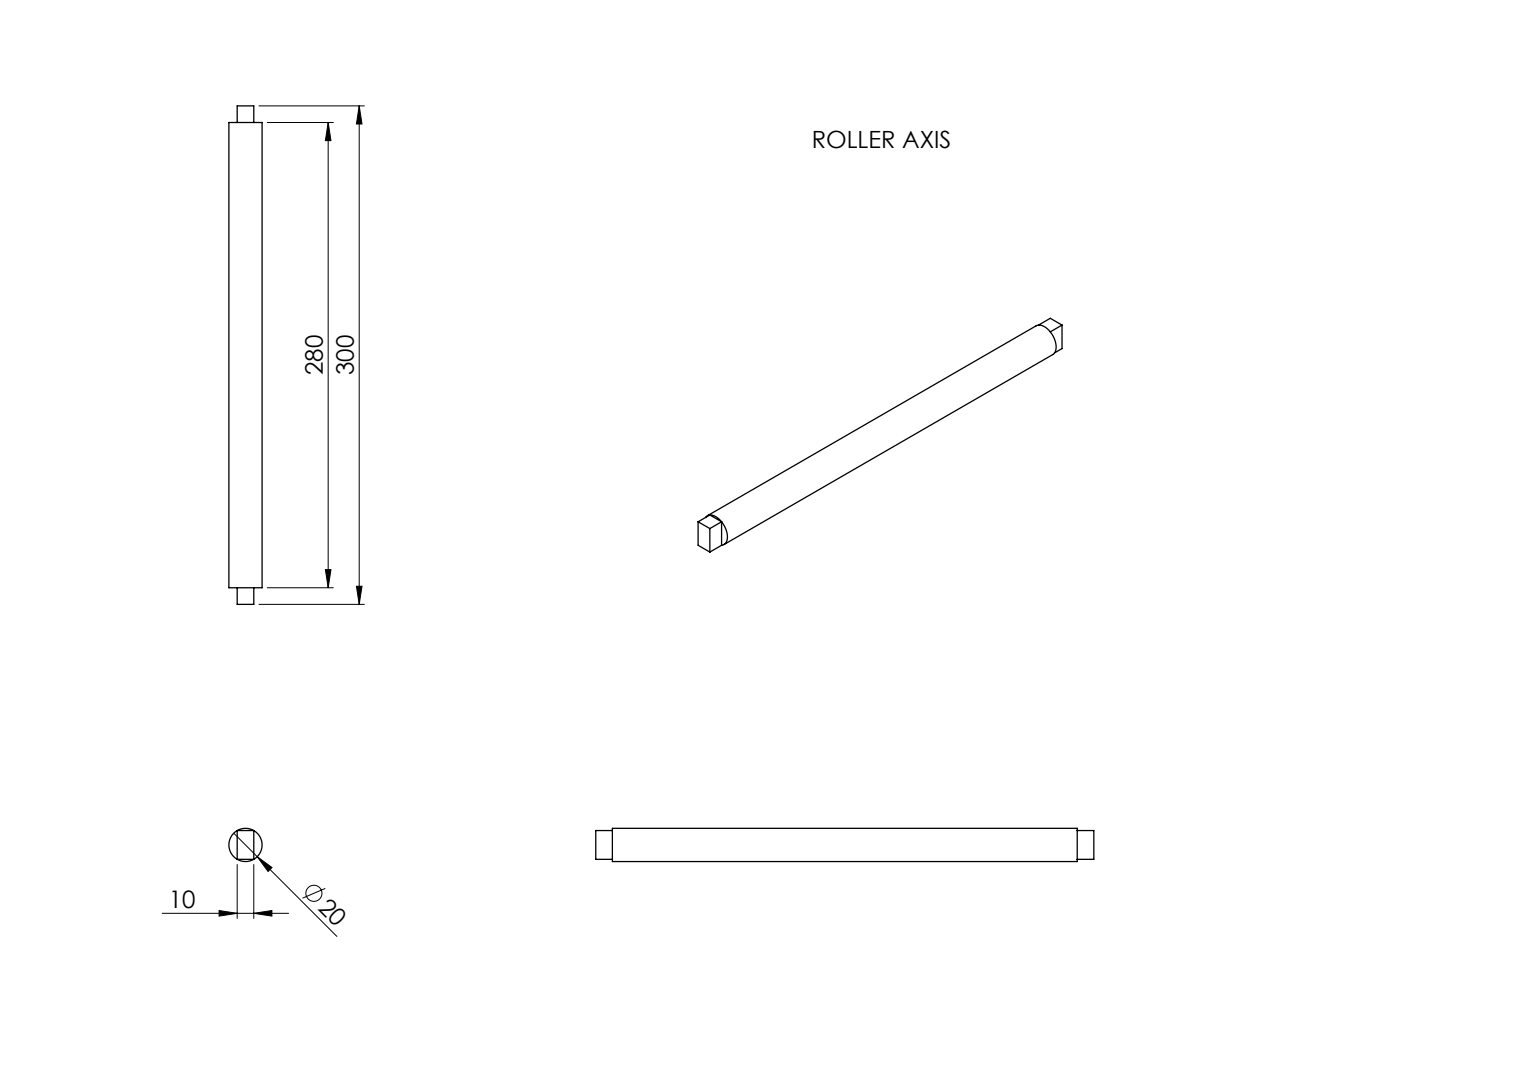
ISO-10303-21;
HEADER;
FILE_DESCRIPTION (('STEP AP214'),
    '1' );
FILE_NAME ('roller axis.step',
    '2026-10-24T14:05:44',
    ( '' ),
    ( '' ),
    'SwSTEP 2.0',
    'SolidWorks 2026',
    '' );
FILE_SCHEMA (( 'AUTOMOTIVE_DESIGN' ));
ENDSEC;

DATA;
#12=PLANE ( 'NONE',  #5087 ) ;
#25=ORIENTED_EDGE ( 'NONE', *, *, #1141, .F. ) ;
#27=CARTESIAN_POINT ( 'NONE',  ( 0.000000000000000000, 0.000000000000000000, 140.0000000000000000 ) ) ;
#37=FILL_AREA_STYLE_COLOUR ( '', #3895 ) ;
#41=AXIS2_PLACEMENT_3D ( 'NONE', #7313, #7278, #7239 ) ;
#47=FACE_OUTER_BOUND ( 'NONE', #4847, .T. ) ;
#52=DIRECTION ( 'NONE',  ( 0.000000000000000000, -0.000000000000000000, 1.000000000000000000 ) ) ;
#53=CARTESIAN_POINT ( 'NONE',  ( 4.999999999999997335, -8.660254037844389075, -140.0000000000000000 ) ) ;
#72=ORIENTED_EDGE ( 'NONE', *, *, #5764, .T. ) ;
#80=CARTESIAN_POINT ( 'NONE',  ( -5.000000000000000888, 8.660254037844390851, 150.0000000000000000 ) ) ;
#83=DIRECTION ( 'NONE',  ( 1.000000000000000000, 0.000000000000000000, -0.000000000000000000 ) ) ;
#94=ADVANCED_FACE ( 'NONE', ( #3566 ), #5869, .F. ) ;
#97=DIRECTION ( 'NONE',  ( 1.000000000000000000, 0.000000000000000000, -0.000000000000000000 ) ) ;
#100=LINE ( 'NONE', #5559, #7316 ) ;
#117=PLANE ( 'NONE',  #3650 ) ;
#124=ORIENTED_EDGE ( 'NONE', *, *, #2636, .T. ) ;
#128=PLANE ( 'NONE',  #3351 ) ;
#140=EDGE_LOOP ( 'NONE', ( #451, #3034, #5054, #639, #3841, #3880, #6414, #6214 ) ) ;
#149=CARTESIAN_POINT ( 'NONE',  ( -5.000000000000000888, -8.660254037844389075, -150.0000000000000000 ) ) ;
#172=DIRECTION ( 'NONE',  ( -1.000000000000000000, 0.000000000000000000, 0.000000000000000000 ) ) ;
#174=ORIENTED_EDGE ( 'NONE', *, *, #1060, .T. ) ;
#181=CIRCLE ( 'NONE', #4359, 10.00000000000000000 ) ;
#189=CARTESIAN_POINT ( 'NONE',  ( 4.999999999999999112, 8.660254037844390851, 150.0000000000000000 ) ) ;
#191=FACE_OUTER_BOUND ( 'NONE', #1286, .T. ) ;
#199=ORIENTED_EDGE ( 'NONE', *, *, #1070, .F. ) ;
#205=ADVANCED_FACE ( 'NONE', ( #4414 ), #1489, .F. ) ;
#217=ORIENTED_EDGE ( 'NONE', *, *, #4171, .T. ) ;
#221=DIRECTION ( 'NONE',  ( 0.000000000000000000, -1.000000000000000000, 0.000000000000000000 ) ) ;
#252=ORIENTED_EDGE ( 'NONE', *, *, #6107, .T. ) ;
#256=AXIS2_PLACEMENT_3D ( 'NONE', #4917, #1432, #2617 ) ;
#292=ORIENTED_EDGE ( 'NONE', *, *, #3168, .F. ) ;
#300=ORIENTED_EDGE ( 'NONE', *, *, #2593, .F. ) ;
#328=DIRECTION ( 'NONE',  ( 1.000000000000000000, 0.000000000000000000, 0.000000000000000000 ) ) ;
#331=ADVANCED_FACE ( 'NONE', ( #6163 ), #6723, .T. ) ;
#352=CYLINDRICAL_SURFACE ( 'NONE', #41, 10.00000000000000000 ) ;
#359=DIRECTION ( 'NONE',  ( -0.000000000000000000, -0.000000000000000000, -1.000000000000000000 ) ) ;
#360=ORIENTED_EDGE ( 'NONE', *, *, #1641, .T. ) ;
#363=FACE_OUTER_BOUND ( 'NONE', #5495, .T. ) ;
#384=ORIENTED_EDGE ( 'NONE', *, *, #3152, .F. ) ;
#392=FACE_OUTER_BOUND ( 'NONE', #2164, .T. ) ;
#397=FACE_OUTER_BOUND ( 'NONE', #140, .T. ) ;
#422=CARTESIAN_POINT ( 'NONE',  ( -5.000000000000000888, -8.660254037844389075, -140.0000000000000284 ) ) ;
#424=CARTESIAN_POINT ( 'NONE',  ( -10.00000000000000000, 0.000000000000000000, -140.0000000000000000 ) ) ;
#426=ORIENTED_EDGE ( 'NONE', *, *, #4897, .F. ) ;
#451=ORIENTED_EDGE ( 'NONE', *, *, #5219, .F. ) ;
#454=EDGE_LOOP ( 'NONE', ( #6459, #72, #5565, #1387 ) ) ;
#456=DIRECTION ( 'NONE',  ( 1.000000000000000000, 0.000000000000000000, -0.000000000000000000 ) ) ;
#457=CARTESIAN_POINT ( 'NONE',  ( -5.000000000000000888, 8.660254037844390851, -150.0000000000000000 ) ) ;
#476=ORIENTED_EDGE ( 'NONE', *, *, #4916, .F. ) ;
#477=LINE ( 'NONE', #3366, #540 ) ;
#537=AXIS2_PLACEMENT_3D ( 'NONE', #2124, #3352, #7303 ) ;
#540=VECTOR ( 'NONE', #6836, 1000.000000000000000 ) ;
#568=DIRECTION ( 'NONE',  ( 1.000000000000000000, 0.000000000000000000, 0.000000000000000000 ) ) ;
#569=AXIS2_PLACEMENT_3D ( 'NONE', #2262, #6216, #568 ) ;
#572=CARTESIAN_POINT ( 'NONE',  ( -5.000000000000000888, 8.660254037844390851, 150.0000000000000000 ) ) ;
#590=CARTESIAN_POINT ( 'NONE',  ( 4.999999999999999112, 8.660254037844390851, -150.0000000000000000 ) ) ;
#597=CARTESIAN_POINT ( 'NONE',  ( -5.000000000000000888, 0.000000000000000000, 140.0000000000000000 ) ) ;
#609=LINE ( 'NONE', #1723, #1679 ) ;
#611=CARTESIAN_POINT ( 'NONE',  ( -5.000000000000000888, -8.660254037844389075, 150.0000000000000000 ) ) ;
#613=ADVANCED_FACE ( 'NONE', ( #47 ), #1091, .F. ) ;
#627=ADVANCED_FACE ( 'NONE', ( #4608 ), #12, .F. ) ;
#628=DIRECTION ( 'NONE',  ( 0.000000000000000000, 0.000000000000000000, 1.000000000000000000 ) ) ;
#630=VERTEX_POINT ( 'NONE', #2832 ) ;
#633=CARTESIAN_POINT ( 'NONE',  ( 0.000000000000000000, 0.000000000000000000, 140.0000000000000000 ) ) ;
#634=LINE ( 'NONE', #149, #4836 ) ;
#639=ORIENTED_EDGE ( 'NONE', *, *, #6547, .F. ) ;
#640=AXIS2_PLACEMENT_3D ( 'NONE', #2848, #6942, #1184 ) ;
#650=AXIS2_PLACEMENT_3D ( 'NONE', #2212, #6051, #988 ) ;
#660=EDGE_CURVE ( 'NONE', #6352, #1004, #181, .T. ) ;
#667=EDGE_LOOP ( 'NONE', ( #840, #4739, #1362, #2962 ) ) ;
#670=STYLED_ITEM ( 'NONE', ( #5899 ), #1370 ) ;
#671=ORIENTED_EDGE ( 'NONE', *, *, #5764, .F. ) ;
#689=ORIENTED_EDGE ( 'NONE', *, *, #5366, .F. ) ;
#692=DIRECTION ( 'NONE',  ( 0.000000000000000000, 0.000000000000000000, 1.000000000000000000 ) ) ;
#740=ADVANCED_FACE ( 'NONE', ( #1129 ), #5700, .F. ) ;
#755=AXIS2_PLACEMENT_3D ( 'NONE', #1285, #4088, #6492 ) ;
#783=ORIENTED_EDGE ( 'NONE', *, *, #4897, .T. ) ;
#794=MANIFOLD_SOLID_BREP ( 'Boss-Extrude2', #5074 ) ;
#820=LINE ( 'NONE', #2560, #5650 ) ;
#832=ADVANCED_FACE ( 'NONE', ( #191 ), #117, .T. ) ;
#840=ORIENTED_EDGE ( 'NONE', *, *, #4441, .F. ) ;
#862=CARTESIAN_POINT ( 'NONE',  ( 0.000000000000000000, 0.000000000000000000, 150.0000000000000000 ) ) ;
#876=CARTESIAN_POINT ( 'NONE',  ( 0.000000000000000000, 8.660254037844390851, -140.0000000000000000 ) ) ;
#901=CARTESIAN_POINT ( 'NONE',  ( 10.00000000000000000, 1.224646799147353256E-15, 140.0000000000000000 ) ) ;
#907=PLANE ( 'NONE',  #5104 ) ;
#919=DIRECTION ( 'NONE',  ( 1.000000000000000000, 0.000000000000000000, -0.000000000000000000 ) ) ;
#942=ORIENTED_EDGE ( 'NONE', *, *, #5085, .T. ) ;
#944=CARTESIAN_POINT ( 'NONE',  ( 4.999999999999999112, 8.660254037844390851, 150.0000000000000000 ) ) ;
#981=ORIENTED_EDGE ( 'NONE', *, *, #1995, .F. ) ;
#988=DIRECTION ( 'NONE',  ( 1.000000000000000000, 0.000000000000000000, -0.000000000000000000 ) ) ;
#1004=VERTEX_POINT ( 'NONE', #5611 ) ;
#1008=AXIS2_PLACEMENT_3D ( 'NONE', #4801, #1517, #3094 ) ;
#1051=CARTESIAN_POINT ( 'NONE',  ( 4.999999999999999112, 8.660254037844390851, -150.0000000000000000 ) ) ;
#1060=EDGE_CURVE ( 'NONE', #6894, #5855, #4448, .T. ) ;
#1070=EDGE_CURVE ( 'NONE', #6814, #1780, #4561, .T. ) ;
#1073=EDGE_CURVE ( 'NONE', #7081, #5227, #4988, .T. ) ;
#1083=CARTESIAN_POINT ( 'NONE',  ( 4.999999999999999112, 0.000000000000000000, 140.0000000000000000 ) ) ;
#1091=PLANE ( 'NONE',  #6280 ) ;
#1094=EDGE_CURVE ( 'NONE', #6847, #3802, #5018, .T. ) ;
#1098=DIRECTION ( 'NONE',  ( 1.000000000000000000, 0.000000000000000000, -0.000000000000000000 ) ) ;
#1112=VECTOR ( 'NONE', #5415, 1000.000000000000000 ) ;
#1129=FACE_OUTER_BOUND ( 'NONE', #1317, .T. ) ;
#1132=ORIENTED_EDGE ( 'NONE', *, *, #7005, .F. ) ;
#1141=EDGE_CURVE ( 'NONE', #4157, #630, #4032, .T. ) ;
#1178=CARTESIAN_POINT ( 'NONE',  ( -5.000000000000000888, 8.660254037844390851, 150.0000000000000000 ) ) ;
#1184=DIRECTION ( 'NONE',  ( 1.000000000000000000, 0.000000000000000000, 0.000000000000000000 ) ) ;
#1189=EDGE_CURVE ( 'NONE', #2308, #3238, #6358, .T. ) ;
#1193=SHAPE_REPRESENTATION ( 'roller axis', ( #1963 ), #5205 ) ;
#1199=DIRECTION ( 'NONE',  ( 0.000000000000000000, -1.000000000000000000, 0.000000000000000000 ) ) ;
#1204=FACE_OUTER_BOUND ( 'NONE', #2091, .T. ) ;
#1208=LINE ( 'NONE', #1178, #5962 ) ;
#1219=ORIENTED_EDGE ( 'NONE', *, *, #1141, .T. ) ;
#1228=DIRECTION ( 'NONE',  ( 0.000000000000000000, -0.000000000000000000, 1.000000000000000000 ) ) ;
#1249=LINE ( 'NONE', #6980, #6621 ) ;
#1285=CARTESIAN_POINT ( 'NONE',  ( 0.000000000000000000, 0.000000000000000000, -140.0000000000000000 ) ) ;
#1286=EDGE_LOOP ( 'NONE', ( #2523, #5606 ) ) ;
#1294=CARTESIAN_POINT ( 'NONE',  ( -5.000000000000000888, -8.660254037844389075, 150.0000000000000000 ) ) ;
#1299=DIRECTION ( 'NONE',  ( 0.000000000000000000, 1.000000000000000000, 0.000000000000000000 ) ) ;
#1317=EDGE_LOOP ( 'NONE', ( #6784, #6485, #783, #2163 ) ) ;
#1327=ORIENTED_EDGE ( 'NONE', *, *, #2416, .F. ) ;
#1329=AXIS2_PLACEMENT_3D ( 'NONE', #611, #5171, #52 ) ;
#1342=PRODUCT_DEFINITION_SHAPE ( 'NONE', 'NONE',  #6666 ) ;
#1352=ADVANCED_FACE ( 'NONE', ( #363 ), #4845, .F. ) ;
#1362=ORIENTED_EDGE ( 'NONE', *, *, #6828, .F. ) ;
#1364=EDGE_CURVE ( 'NONE', #2884, #6814, #4018, .T. ) ;
#1370=ADVANCED_BREP_SHAPE_REPRESENTATION ( '', ( #794, #1963 ), #5205 ) ;
#1376=( NAMED_UNIT ( * ) SI_UNIT ( $, .STERADIAN. ) SOLID_ANGLE_UNIT ( ) );
#1385=VECTOR ( 'NONE', #6183, 1000.000000000000000 ) ;
#1387=ORIENTED_EDGE ( 'NONE', *, *, #4449, .T. ) ;
#1432=DIRECTION ( 'NONE',  ( -0.000000000000000000, -0.000000000000000000, -1.000000000000000000 ) ) ;
#1471=CARTESIAN_POINT ( 'NONE',  ( -5.000000000000000888, -8.660254037844389075, 150.0000000000000000 ) ) ;
#1489=PLANE ( 'NONE',  #5904 ) ;
#1517=DIRECTION ( 'NONE',  ( 0.000000000000000000, 0.000000000000000000, 1.000000000000000000 ) ) ;
#1542=CARTESIAN_POINT ( 'NONE',  ( -5.000000000000000888, -8.660254037844389075, 150.0000000000000000 ) ) ;
#1548=CARTESIAN_POINT ( 'NONE',  ( 0.000000000000000000, 0.000000000000000000, -150.0000000000000000 ) ) ;
#1550=VERTEX_POINT ( 'NONE', #3299 ) ;
#1553=DIRECTION ( 'NONE',  ( 0.000000000000000000, -1.000000000000000000, 0.000000000000000000 ) ) ;
#1560=ORIENTED_EDGE ( 'NONE', *, *, #1073, .F. ) ;
#1570=PLANE ( 'NONE',  #537 ) ;
#1641=EDGE_CURVE ( 'NONE', #6814, #630, #6528, .T. ) ;
#1648=ORIENTED_EDGE ( 'NONE', *, *, #3152, .T. ) ;
#1679=VECTOR ( 'NONE', #4012, 1000.000000000000000 ) ;
#1719=CARTESIAN_POINT ( 'NONE',  ( -5.000000000000000888, -8.660254037844389075, 150.0000000000000000 ) ) ;
#1723=CARTESIAN_POINT ( 'NONE',  ( 10.00000000000000000, 1.224646799147353256E-15, 140.0000000000000000 ) ) ;
#1727=VECTOR ( 'NONE', #5465, 1000.000000000000000 ) ;
#1735=DIRECTION ( 'NONE',  ( 0.000000000000000000, 0.000000000000000000, 1.000000000000000000 ) ) ;
#1743=ADVANCED_FACE ( 'NONE', ( #4907 ), #907, .T. ) ;
#1747=( NAMED_UNIT ( * ) SI_UNIT ( $, .STERADIAN. ) SOLID_ANGLE_UNIT ( ) );
#1760=PLANE ( 'NONE',  #4967 ) ;
#1765=DIRECTION ( 'NONE',  ( 1.000000000000000000, 0.000000000000000000, 0.000000000000000000 ) ) ;
#1780=VERTEX_POINT ( 'NONE', #4271 ) ;
#1911=ORIENTED_EDGE ( 'NONE', *, *, #6967, .T. ) ;
#1963=AXIS2_PLACEMENT_3D ( 'NONE', #2294, #628, #5829 ) ;
#1989=DIRECTION ( 'NONE',  ( 1.000000000000000000, 0.000000000000000000, -0.000000000000000000 ) ) ;
#1994=CARTESIAN_POINT ( 'NONE',  ( 4.999999999999999112, -8.660254037844389075, -150.0000000000000000 ) ) ;
#1995=EDGE_CURVE ( 'NONE', #5227, #6735, #2563, .T. ) ;
#2008=ORIENTED_EDGE ( 'NONE', *, *, #5138, .T. ) ;
#2091=EDGE_LOOP ( 'NONE', ( #5202, #2859, #2616, #7285 ) ) ;
#2115=EDGE_LOOP ( 'NONE', ( #6569, #2579, #4972 ) ) ;
#2124=CARTESIAN_POINT ( 'NONE',  ( -5.000000000000000888, 8.660254037844390851, 150.0000000000000000 ) ) ;
#2163=ORIENTED_EDGE ( 'NONE', *, *, #7005, .T. ) ;
#2164=EDGE_LOOP ( 'NONE', ( #671, #1560 ) ) ;
#2206=LINE ( 'NONE', #7310, #2963 ) ;
#2212=CARTESIAN_POINT ( 'NONE',  ( 0.000000000000000000, 0.000000000000000000, 140.0000000000000000 ) ) ;
#2246=DIRECTION ( 'NONE',  ( 0.000000000000000000, 0.000000000000000000, 1.000000000000000000 ) ) ;
#2262=CARTESIAN_POINT ( 'NONE',  ( 0.000000000000000000, 0.000000000000000000, -140.0000000000000000 ) ) ;
#2274=DIRECTION ( 'NONE',  ( 0.000000000000000000, 0.000000000000000000, 1.000000000000000000 ) ) ;
#2277=CARTESIAN_POINT ( 'NONE',  ( 0.000000000000000000, 0.000000000000000000, -140.0000000000000000 ) ) ;
#2282=ORIENTED_EDGE ( 'NONE', *, *, #4441, .T. ) ;
#2289=EDGE_CURVE ( 'NONE', #6735, #5434, #5541, .T. ) ;
#2293=ORIENTED_EDGE ( 'NONE', *, *, #1094, .F. ) ;
#2294=CARTESIAN_POINT ( 'NONE',  ( 0.000000000000000000, 0.000000000000000000, 0.000000000000000000 ) ) ;
#2308=VERTEX_POINT ( 'NONE', #1471 ) ;
#2349=ORIENTED_EDGE ( 'NONE', *, *, #1070, .T. ) ;
#2400=DIRECTION ( 'NONE',  ( 1.000000000000000000, 0.000000000000000000, -0.000000000000000000 ) ) ;
#2416=EDGE_CURVE ( 'NONE', #1550, #6735, #5364, .T. ) ;
#2426=DIRECTION ( 'NONE',  ( 0.000000000000000000, 0.000000000000000000, 1.000000000000000000 ) ) ;
#2469=PRODUCT ( 'roller axis', 'roller axis', '', ( #3485 ) ) ;
#2487=ADVANCED_FACE ( 'NONE', ( #392 ), #6052, .F. ) ;
#2518=EDGE_LOOP ( 'NONE', ( #360, #2282 ) ) ;
#2522=DIRECTION ( 'NONE',  ( 0.000000000000000000, 0.000000000000000000, 1.000000000000000000 ) ) ;
#2523=ORIENTED_EDGE ( 'NONE', *, *, #3458, .T. ) ;
#2541=ADVANCED_FACE ( 'NONE', ( #6567 ), #7199, .F. ) ;
#2560=CARTESIAN_POINT ( 'NONE',  ( 0.000000000000000000, -8.660254037844389075, -140.0000000000000000 ) ) ;
#2563=CIRCLE ( 'NONE', #3526, 10.00000000000000000 ) ;
#2579=ORIENTED_EDGE ( 'NONE', *, *, #6613, .F. ) ;
#2593=EDGE_CURVE ( 'NONE', #2887, #6814, #477, .T. ) ;
#2598=DIRECTION ( 'NONE',  ( -1.000000000000000000, 0.000000000000000000, 0.000000000000000000 ) ) ;
#2601=DIRECTION ( 'NONE',  ( 1.000000000000000000, 0.000000000000000000, 0.000000000000000000 ) ) ;
#2616=ORIENTED_EDGE ( 'NONE', *, *, #1189, .F. ) ;
#2617=DIRECTION ( 'NONE',  ( -1.000000000000000000, 0.000000000000000000, 0.000000000000000000 ) ) ;
#2624=CARTESIAN_POINT ( 'NONE',  ( -5.000000000000000888, 8.660254037844390851, 150.0000000000000000 ) ) ;
#2631=LINE ( 'NONE', #7140, #5691 ) ;
#2636=EDGE_CURVE ( 'NONE', #5227, #6847, #1208, .T. ) ;
#2648=LINE ( 'NONE', #1542, #2756 ) ;
#2686=VECTOR ( 'NONE', #2828, 1000.000000000000000 ) ;
#2693=EDGE_LOOP ( 'NONE', ( #6432, #7023, #1911, #5734 ) ) ;
#2700=DIRECTION ( 'NONE',  ( 1.000000000000000000, 0.000000000000000000, -0.000000000000000000 ) ) ;
#2739=CARTESIAN_POINT ( 'NONE',  ( 0.000000000000000000, 0.000000000000000000, 140.0000000000000000 ) ) ;
#2742=LINE ( 'NONE', #876, #4439 ) ;
#2756=VECTOR ( 'NONE', #4425, 1000.000000000000000 ) ;
#2761=CARTESIAN_POINT ( 'NONE',  ( 0.000000000000000000, 0.000000000000000000, -140.0000000000000000 ) ) ;
#2790=DIRECTION ( 'NONE',  ( 0.000000000000000000, -1.000000000000000000, 0.000000000000000000 ) ) ;
#2828=DIRECTION ( 'NONE',  ( -1.000000000000000000, -0.000000000000000000, -0.000000000000000000 ) ) ;
#2832=CARTESIAN_POINT ( 'NONE',  ( -5.000000000000000888, 8.660254037844390851, 140.0000000000000000 ) ) ;
#2848=CARTESIAN_POINT ( 'NONE',  ( 0.000000000000000000, 0.000000000000000000, 140.0000000000000000 ) ) ;
#2852=DIRECTION ( 'NONE',  ( 0.000000000000000000, -1.000000000000000000, 0.000000000000000000 ) ) ;
#2856=CARTESIAN_POINT ( 'NONE',  ( -5.000000000000000888, 8.660254037844390851, -150.0000000000000000 ) ) ;
#2859=ORIENTED_EDGE ( 'NONE', *, *, #6351, .F. ) ;
#2860=DIRECTION ( 'NONE',  ( -1.000000000000000000, 0.000000000000000000, 0.000000000000000000 ) ) ;
#2863=ORIENTED_EDGE ( 'NONE', *, *, #6967, .F. ) ;
#2865=CARTESIAN_POINT ( 'NONE',  ( -5.000000000000000888, 8.660254037844387298, -140.0000000000000000 ) ) ;
#2884=VERTEX_POINT ( 'NONE', #901 ) ;
#2887=VERTEX_POINT ( 'NONE', #5536 ) ;
#2893=DIRECTION ( 'NONE',  ( 1.000000000000000000, 0.000000000000000000, 0.000000000000000000 ) ) ;
#2897=EDGE_LOOP ( 'NONE', ( #1648, #6143, #1219 ) ) ;
#2906=MECHANICAL_DESIGN_GEOMETRIC_PRESENTATION_REPRESENTATION('',(#670),#4713);
#2962=ORIENTED_EDGE ( 'NONE', *, *, #2593, .T. ) ;
#2963=VECTOR ( 'NONE', #6309, 1000.000000000000000 ) ;
#2979=AXIS2_PLACEMENT_3D ( 'NONE', #2739, #1735, #4517 ) ;
#3034=ORIENTED_EDGE ( 'NONE', *, *, #5138, .F. ) ;
#3037=VECTOR ( 'NONE', #6952, 1000.000000000000000 ) ;
#3094=DIRECTION ( 'NONE',  ( 1.000000000000000000, 0.000000000000000000, 0.000000000000000000 ) ) ;
#3115=ORIENTED_EDGE ( 'NONE', *, *, #1364, .F. ) ;
#3124=VECTOR ( 'NONE', #359, 1000.000000000000000 ) ;
#3150=AXIS2_PLACEMENT_3D ( 'NONE', #2624, #1989, #6063 ) ;
#3152=EDGE_CURVE ( 'NONE', #630, #1550, #5065, .T. ) ;
#3167=CARTESIAN_POINT ( 'NONE',  ( 0.000000000000000000, 0.000000000000000000, -140.0000000000000000 ) ) ;
#3168=EDGE_CURVE ( 'NONE', #3238, #2887, #6917, .T. ) ;
#3188=LINE ( 'NONE', #4294, #1112 ) ;
#3232=EDGE_CURVE ( 'NONE', #5434, #6352, #4697, .T. ) ;
#3238=VERTEX_POINT ( 'NONE', #7022 ) ;
#3273=EDGE_CURVE ( 'NONE', #1780, #4157, #1249, .T. ) ;
#3299=CARTESIAN_POINT ( 'NONE',  ( -10.00000000000000000, 0.000000000000000000, 140.0000000000000000 ) ) ;
#3336=CARTESIAN_POINT ( 'NONE',  ( -4.999999999999997335, -8.660254037844389075, 140.0000000000000000 ) ) ;
#3351=AXIS2_PLACEMENT_3D ( 'NONE', #5322, #97, #3515 ) ;
#3352=DIRECTION ( 'NONE',  ( 0.000000000000000000, -1.000000000000000000, 0.000000000000000000 ) ) ;
#3366=CARTESIAN_POINT ( 'NONE',  ( 4.999999999999999112, 8.660254037844390851, 150.0000000000000000 ) ) ;
#3439=PLANE ( 'NONE',  #1329 ) ;
#3443=DIRECTION ( 'NONE',  ( -0.000000000000000000, -0.000000000000000000, -1.000000000000000000 ) ) ;
#3454=SURFACE_STYLE_FILL_AREA ( #3561 ) ;
#3458=EDGE_CURVE ( 'NONE', #4157, #1780, #7202, .T. ) ;
#3471=PLANE ( 'NONE',  #4280 ) ;
#3485=PRODUCT_CONTEXT ( 'NONE', #3717, 'mechanical' ) ;
#3491=PLANE ( 'NONE',  #6961 ) ;
#3515=DIRECTION ( 'NONE',  ( -0.000000000000000000, 0.000000000000000000, -1.000000000000000000 ) ) ;
#3526=AXIS2_PLACEMENT_3D ( 'NONE', #4013, #5140, #5841 ) ;
#3528=ORIENTED_EDGE ( 'NONE', *, *, #2289, .F. ) ;
#3561=FILL_AREA_STYLE ('',( #37 ) ) ;
#3566=FACE_OUTER_BOUND ( 'NONE', #6734, .T. ) ;
#3567=( NAMED_UNIT ( * ) PLANE_ANGLE_UNIT ( ) SI_UNIT ( $, .RADIAN. ) );
#3649=ADVANCED_FACE ( 'NONE', ( #3700 ), #352, .T. ) ;
#3650=AXIS2_PLACEMENT_3D ( 'NONE', #4177, #6364, #83 ) ;
#3700=FACE_OUTER_BOUND ( 'NONE', #4683, .T. ) ;
#3717=APPLICATION_CONTEXT ( 'automotive_design' ) ;
#3774=VECTOR ( 'NONE', #2852, 1000.000000000000000 ) ;
#3802=VERTEX_POINT ( 'NONE', #4509 ) ;
#3822=CARTESIAN_POINT ( 'NONE',  ( -5.000000000000000888, 0.000000000000000000, -140.0000000000000000 ) ) ;
#3824=DIRECTION ( 'NONE',  ( 1.000000000000000000, 0.000000000000000000, 0.000000000000000000 ) ) ;
#3834=ADVANCED_FACE ( 'NONE', ( #1204 ), #3439, .F. ) ;
#3841=ORIENTED_EDGE ( 'NONE', *, *, #2416, .T. ) ;
#3872=PRODUCT_DEFINITION_FORMATION_WITH_SPECIFIED_SOURCE ( 'ANY', '', #2469, .NOT_KNOWN. ) ;
#3880=ORIENTED_EDGE ( 'NONE', *, *, #2289, .T. ) ;
#3893=CARTESIAN_POINT ( 'NONE',  ( 4.999999999999999112, 8.660254037844390851, 140.0000000000000000 ) ) ;
#3895=COLOUR_RGB ( '',0.8941176470588234615, 0.8941176470588234615, 0.8941176470588234615 ) ;
#3900=ORIENTED_EDGE ( 'NONE', *, *, #1094, .T. ) ;
#3907=FACE_OUTER_BOUND ( 'NONE', #2115, .T. ) ;
#3911=( GEOMETRIC_REPRESENTATION_CONTEXT ( 3 ) GLOBAL_UNCERTAINTY_ASSIGNED_CONTEXT ( ( #4933 ) ) GLOBAL_UNIT_ASSIGNED_CONTEXT ( ( #4749, #3567, #1376 ) ) REPRESENTATION_CONTEXT ( 'NONE', 'WORKASPACE' ) );
#3958=AXIS2_PLACEMENT_3D ( 'NONE', #6227, #2274, #6197 ) ;
#3968=FACE_OUTER_BOUND ( 'NONE', #667, .T. ) ;
#3979=DIRECTION ( 'NONE',  ( -0.000000000000000000, -0.000000000000000000, -1.000000000000000000 ) ) ;
#4008=AXIS2_PLACEMENT_3D ( 'NONE', #6481, #5920, #4077 ) ;
#4012=DIRECTION ( 'NONE',  ( -0.000000000000000000, -0.000000000000000000, -1.000000000000000000 ) ) ;
#4013=CARTESIAN_POINT ( 'NONE',  ( 0.000000000000000000, 0.000000000000000000, -140.0000000000000000 ) ) ;
#4018=CIRCLE ( 'NONE', #5570, 10.00000000000000000 ) ;
#4032=LINE ( 'NONE', #597, #1385 ) ;
#4038=PLANE ( 'NONE',  #2979 ) ;
#4077=DIRECTION ( 'NONE',  ( 1.000000000000000000, 0.000000000000000000, 0.000000000000000000 ) ) ;
#4088=DIRECTION ( 'NONE',  ( 0.000000000000000000, 0.000000000000000000, 1.000000000000000000 ) ) ;
#4110=AXIS2_PLACEMENT_3D ( 'NONE', #1719, #1299, #1228 ) ;
#4138=( LENGTH_UNIT ( ) NAMED_UNIT ( * ) SI_UNIT ( .MILLI., .METRE. ) );
#4157=VERTEX_POINT ( 'NONE', #3336 ) ;
#4171=EDGE_CURVE ( 'NONE', #7081, #6352, #7066, .T. ) ;
#4177=CARTESIAN_POINT ( 'NONE',  ( 0.000000000000000000, 0.000000000000000000, 140.0000000000000000 ) ) ;
#4248=CARTESIAN_POINT ( 'NONE',  ( 0.000000000000000000, 0.000000000000000000, 140.0000000000000000 ) ) ;
#4271=CARTESIAN_POINT ( 'NONE',  ( 4.999999999999999112, -8.660254037844389075, 140.0000000000000000 ) ) ;
#4280=AXIS2_PLACEMENT_3D ( 'NONE', #5771, #2246, #1098 ) ;
#4294=CARTESIAN_POINT ( 'NONE',  ( -5.000000000000000888, -8.660254037844389075, 150.0000000000000000 ) ) ;
#4307=DIRECTION ( 'NONE',  ( 1.000000000000000000, 0.000000000000000000, 0.000000000000000000 ) ) ;
#4315=VECTOR ( 'NONE', #4391, 1000.000000000000000 ) ;
#4331=ORIENTED_EDGE ( 'NONE', *, *, #1364, .T. ) ;
#4344=AXIS2_PLACEMENT_3D ( 'NONE', #189, #4748, #7034 ) ;
#4359=AXIS2_PLACEMENT_3D ( 'NONE', #2761, #6649, #2893 ) ;
#4391=DIRECTION ( 'NONE',  ( -0.000000000000000000, -0.000000000000000000, -1.000000000000000000 ) ) ;
#4398=DIRECTION ( 'NONE',  ( 0.000000000000000000, 0.000000000000000000, 1.000000000000000000 ) ) ;
#4410=ORIENTED_EDGE ( 'NONE', *, *, #5435, .F. ) ;
#4414=FACE_OUTER_BOUND ( 'NONE', #4976, .T. ) ;
#4416=EDGE_LOOP ( 'NONE', ( #2008, #4331, #2349 ) ) ;
#4425=DIRECTION ( 'NONE',  ( -0.000000000000000000, -0.000000000000000000, -1.000000000000000000 ) ) ;
#4433=EDGE_LOOP ( 'NONE', ( #4672, #1132, #2293, #5210 ) ) ;
#4439=VECTOR ( 'NONE', #919, 1000.000000000000000 ) ;
#4440=VECTOR ( 'NONE', #1553, 1000.000000000000000 ) ;
#4441=EDGE_CURVE ( 'NONE', #630, #6814, #6281, .T. ) ;
#4448=LINE ( 'NONE', #1051, #7015 ) ;
#4449=EDGE_CURVE ( 'NONE', #5855, #6847, #100, .T. ) ;
#4475=CARTESIAN_POINT ( 'NONE',  ( 4.999999999999999112, 0.000000000000000000, -140.0000000000000000 ) ) ;
#4509=CARTESIAN_POINT ( 'NONE',  ( -5.000000000000000888, -8.660254037844389075, -150.0000000000000000 ) ) ;
#4517=DIRECTION ( 'NONE',  ( 1.000000000000000000, 0.000000000000000000, -0.000000000000000000 ) ) ;
#4545=ADVANCED_FACE ( 'NONE', ( #397 ), #4963, .T. ) ;
#4555=CIRCLE ( 'NONE', #3958, 10.00000000000000000 ) ;
#4561=LINE ( 'NONE', #1083, #3774 ) ;
#4575=DIRECTION ( 'NONE',  ( 0.000000000000000000, 0.000000000000000000, 1.000000000000000000 ) ) ;
#4594=( NAMED_UNIT ( * ) SI_UNIT ( $, .STERADIAN. ) SOLID_ANGLE_UNIT ( ) );
#4598=DIRECTION ( 'NONE',  ( -0.000000000000000000, 1.000000000000000000, -0.000000000000000000 ) ) ;
#4608=FACE_OUTER_BOUND ( 'NONE', #454, .T. ) ;
#4654=ADVANCED_FACE ( 'NONE', ( #7322 ), #4038, .T. ) ;
#4660=SURFACE_STYLE_USAGE ( .BOTH. , #5792 ) ;
#4666=DIRECTION ( 'NONE',  ( 1.000000000000000000, 0.000000000000000000, 0.000000000000000000 ) ) ;
#4672=ORIENTED_EDGE ( 'NONE', *, *, #1060, .F. ) ;
#4679=ORIENTED_EDGE ( 'NONE', *, *, #6613, .T. ) ;
#4683=EDGE_LOOP ( 'NONE', ( #3115, #4866, #4679, #6439, #6225, #1327, #384, #7301 ) ) ;
#4697=CIRCLE ( 'NONE', #755, 10.00000000000000000 ) ;
#4713=( GEOMETRIC_REPRESENTATION_CONTEXT ( 3 ) GLOBAL_UNCERTAINTY_ASSIGNED_CONTEXT ( ( #7062 ) ) GLOBAL_UNIT_ASSIGNED_CONTEXT ( ( #4138, #6464, #4594 ) ) REPRESENTATION_CONTEXT ( 'NONE', 'WORKASPACE' ) );
#4739=ORIENTED_EDGE ( 'NONE', *, *, #7160, .F. ) ;
#4748=DIRECTION ( 'NONE',  ( -1.000000000000000000, 0.000000000000000000, 0.000000000000000000 ) ) ;
#4749=( LENGTH_UNIT ( ) NAMED_UNIT ( * ) SI_UNIT ( .MILLI., .METRE. ) );
#4762=DIRECTION ( 'NONE',  ( 1.000000000000000000, 0.000000000000000000, 0.000000000000000000 ) ) ;
#4801=CARTESIAN_POINT ( 'NONE',  ( 0.000000000000000000, 0.000000000000000000, -140.0000000000000000 ) ) ;
#4810=DIRECTION ( 'NONE',  ( -0.000000000000000000, -0.000000000000000000, -1.000000000000000000 ) ) ;
#4811=VECTOR ( 'NONE', #5747, 1000.000000000000000 ) ;
#4816=ADVANCED_FACE ( 'NONE', ( #5850 ), #128, .F. ) ;
#4836=VECTOR ( 'NONE', #4666, 1000.000000000000000 ) ;
#4838=ORIENTED_EDGE ( 'NONE', *, *, #3232, .F. ) ;
#4845=PLANE ( 'NONE',  #3150 ) ;
#4847=EDGE_LOOP ( 'NONE', ( #199, #300, #292, #7091 ) ) ;
#4866=ORIENTED_EDGE ( 'NONE', *, *, #5219, .T. ) ;
#4890=CARTESIAN_POINT ( 'NONE',  ( 0.000000000000000000, 0.000000000000000000, -140.0000000000000000 ) ) ;
#4897=EDGE_CURVE ( 'NONE', #5434, #3802, #2648, .T. ) ;
#4907=FACE_OUTER_BOUND ( 'NONE', #2693, .T. ) ;
#4916=EDGE_CURVE ( 'NONE', #7081, #5855, #7276, .T. ) ;
#4917=CARTESIAN_POINT ( 'NONE',  ( 0.000000000000000000, 0.000000000000000000, 140.0000000000000000 ) ) ;
#4933=UNCERTAINTY_MEASURE_WITH_UNIT (LENGTH_MEASURE( 1.000000000000000082E-05 ), #4749, 'distance_accuracy_value', 'NONE');
#4963=CYLINDRICAL_SURFACE ( 'NONE', #256, 10.00000000000000000 ) ;
#4967=AXIS2_PLACEMENT_3D ( 'NONE', #2277, #4575, #6313 ) ;
#4969=AXIS2_PLACEMENT_3D ( 'NONE', #1548, #6088, #3824 ) ;
#4972=ORIENTED_EDGE ( 'NONE', *, *, #660, .F. ) ;
#4976=EDGE_LOOP ( 'NONE', ( #6363, #3528, #981 ) ) ;
#4988=CIRCLE ( 'NONE', #569, 10.00000000000000000 ) ;
#5018=LINE ( 'NONE', #457, #5704 ) ;
#5033=LINE ( 'NONE', #6908, #5921 ) ;
#5054=ORIENTED_EDGE ( 'NONE', *, *, #3458, .F. ) ;
#5065=CIRCLE ( 'NONE', #640, 10.00000000000000000 ) ;
#5074=CLOSED_SHELL ( 'NONE', ( #3649, #4654, #5666, #331, #832, #6368, #2487, #205, #6403, #4545, #2541, #740, #1352, #627, #94, #613, #5494, #4816, #3834, #1743 ) ) ;
#5085=EDGE_CURVE ( 'NONE', #6352, #6894, #2206, .T. ) ;
#5087=AXIS2_PLACEMENT_3D ( 'NONE', #6901, #1199, #6307 ) ;
#5104=AXIS2_PLACEMENT_3D ( 'NONE', #862, #5428, #4307 ) ;
#5120=CARTESIAN_POINT ( 'NONE',  ( 4.999999999999999112, 8.660254037844390851, 150.0000000000000000 ) ) ;
#5136=CARTESIAN_POINT ( 'NONE',  ( 4.999999999999999112, 8.660254037844390851, 150.0000000000000000 ) ) ;
#5138=EDGE_CURVE ( 'NONE', #1780, #2884, #4555, .T. ) ;
#5140=DIRECTION ( 'NONE',  ( 0.000000000000000000, 0.000000000000000000, 1.000000000000000000 ) ) ;
#5171=DIRECTION ( 'NONE',  ( 0.000000000000000000, 1.000000000000000000, 0.000000000000000000 ) ) ;
#5202=ORIENTED_EDGE ( 'NONE', *, *, #3273, .F. ) ;
#5205=( GEOMETRIC_REPRESENTATION_CONTEXT ( 3 ) GLOBAL_UNCERTAINTY_ASSIGNED_CONTEXT ( ( #5336 ) ) GLOBAL_UNIT_ASSIGNED_CONTEXT ( ( #6325, #5295, #1747 ) ) REPRESENTATION_CONTEXT ( 'NONE', 'WORKASPACE' ) );
#5210=ORIENTED_EDGE ( 'NONE', *, *, #4449, .F. ) ;
#5217=DIRECTION ( 'NONE',  ( 1.000000000000000000, 0.000000000000000000, -0.000000000000000000 ) ) ;
#5219=EDGE_CURVE ( 'NONE', #2884, #1004, #609, .T. ) ;
#5227=VERTEX_POINT ( 'NONE', #2865 ) ;
#5295=( NAMED_UNIT ( * ) PLANE_ANGLE_UNIT ( ) SI_UNIT ( $, .RADIAN. ) );
#5315=CIRCLE ( 'NONE', #4008, 10.00000000000000000 ) ;
#5322=CARTESIAN_POINT ( 'NONE',  ( -5.000000000000000888, 8.660254037844390851, 150.0000000000000000 ) ) ;
#5336=UNCERTAINTY_MEASURE_WITH_UNIT (LENGTH_MEASURE( 1.000000000000000082E-05 ), #6325, 'distance_accuracy_value', 'NONE');
#5364=LINE ( 'NONE', #5473, #3124 ) ;
#5366=EDGE_CURVE ( 'NONE', #6352, #5434, #820, .T. ) ;
#5400=DIRECTION ( 'NONE',  ( 0.000000000000000000, 0.000000000000000000, 1.000000000000000000 ) ) ;
#5415=DIRECTION ( 'NONE',  ( -0.000000000000000000, -0.000000000000000000, -1.000000000000000000 ) ) ;
#5428=DIRECTION ( 'NONE',  ( -0.000000000000000000, 0.000000000000000000, 1.000000000000000000 ) ) ;
#5434=VERTEX_POINT ( 'NONE', #422 ) ;
#5435=EDGE_CURVE ( 'NONE', #2308, #4157, #3188, .T. ) ;
#5465=DIRECTION ( 'NONE',  ( -0.000000000000000000, 1.000000000000000000, 0.000000000000000000 ) ) ;
#5473=CARTESIAN_POINT ( 'NONE',  ( -10.00000000000000000, 0.000000000000000000, 140.0000000000000000 ) ) ;
#5475=CARTESIAN_POINT ( 'NONE',  ( -5.000000000000000888, 8.660254037844390851, 150.0000000000000000 ) ) ;
#5494=ADVANCED_FACE ( 'NONE', ( #3968 ), #1570, .F. ) ;
#5495=EDGE_LOOP ( 'NONE', ( #426, #252, #124, #3900 ) ) ;
#5524=AXIS2_PLACEMENT_3D ( 'NONE', #5819, #692, #4762 ) ;
#5536=CARTESIAN_POINT ( 'NONE',  ( 4.999999999999999112, 8.660254037844390851, 150.0000000000000000 ) ) ;
#5541=CIRCLE ( 'NONE', #1008, 10.00000000000000000 ) ;
#5559=CARTESIAN_POINT ( 'NONE',  ( -5.000000000000000888, 8.660254037844390851, -150.0000000000000000 ) ) ;
#5563=AXIS2_PLACEMENT_3D ( 'NONE', #6632, #2522, #2601 ) ;
#5565=ORIENTED_EDGE ( 'NONE', *, *, #4916, .T. ) ;
#5570=AXIS2_PLACEMENT_3D ( 'NONE', #4248, #6541, #328 ) ;
#5573=DIRECTION ( 'NONE',  ( 0.000000000000000000, 0.000000000000000000, 1.000000000000000000 ) ) ;
#5579=LINE ( 'NONE', #572, #2686 ) ;
#5606=ORIENTED_EDGE ( 'NONE', *, *, #3273, .T. ) ;
#5611=CARTESIAN_POINT ( 'NONE',  ( 10.00000000000000000, 1.224646799147353256E-15, -140.0000000000000000 ) ) ;
#5650=VECTOR ( 'NONE', #2598, 1000.000000000000000 ) ;
#5666=ADVANCED_FACE ( 'NONE', ( #5975 ), #3491, .T. ) ;
#5691=VECTOR ( 'NONE', #4810, 1000.000000000000000 ) ;
#5700=PLANE ( 'NONE',  #4110 ) ;
#5704=VECTOR ( 'NONE', #2790, 1000.000000000000000 ) ;
#5716=CARTESIAN_POINT ( 'NONE',  ( 0.000000000000000000, 8.660254037844390851, 140.0000000000000000 ) ) ;
#5734=ORIENTED_EDGE ( 'NONE', *, *, #1189, .T. ) ;
#5747=DIRECTION ( 'NONE',  ( -0.000000000000000000, 1.000000000000000000, -0.000000000000000000 ) ) ;
#5753=SHAPE_REPRESENTATION_RELATIONSHIP ( 'NONE' , 'NONE' ,  #1193, #1370 ) ;
#5764=EDGE_CURVE ( 'NONE', #5227, #7081, #2742, .T. ) ;
#5771=CARTESIAN_POINT ( 'NONE',  ( 0.000000000000000000, 0.000000000000000000, -140.0000000000000000 ) ) ;
#5784=VERTEX_POINT ( 'NONE', #5475 ) ;
#5792=SURFACE_SIDE_STYLE ('',( #3454 ) ) ;
#5796=CIRCLE ( 'NONE', #5563, 10.00000000000000000 ) ;
#5819=CARTESIAN_POINT ( 'NONE',  ( 0.000000000000000000, 0.000000000000000000, 140.0000000000000000 ) ) ;
#5829=DIRECTION ( 'NONE',  ( 1.000000000000000000, 0.000000000000000000, 0.000000000000000000 ) ) ;
#5841=DIRECTION ( 'NONE',  ( 1.000000000000000000, 0.000000000000000000, 0.000000000000000000 ) ) ;
#5850=FACE_OUTER_BOUND ( 'NONE', #6921, .T. ) ;
#5855=VERTEX_POINT ( 'NONE', #590 ) ;
#5869=PLANE ( 'NONE',  #4344 ) ;
#5899=PRESENTATION_STYLE_ASSIGNMENT (( #4660 ) ) ;
#5904=AXIS2_PLACEMENT_3D ( 'NONE', #4890, #5573, #456 ) ;
#5920=DIRECTION ( 'NONE',  ( 0.000000000000000000, 0.000000000000000000, 1.000000000000000000 ) ) ;
#5921=VECTOR ( 'NONE', #3979, 1000.000000000000000 ) ;
#5962=VECTOR ( 'NONE', #3443, 1000.000000000000000 ) ;
#5975=FACE_OUTER_BOUND ( 'NONE', #2518, .T. ) ;
#6003=LINE ( 'NONE', #3822, #1727 ) ;
#6051=DIRECTION ( 'NONE',  ( 0.000000000000000000, 0.000000000000000000, 1.000000000000000000 ) ) ;
#6052=PLANE ( 'NONE',  #6623 ) ;
#6063=DIRECTION ( 'NONE',  ( -0.000000000000000000, 0.000000000000000000, -1.000000000000000000 ) ) ;
#6080=PRODUCT_DEFINITION_CONTEXT ( 'detailed design', #6326, 'design' ) ;
#6088=DIRECTION ( 'NONE',  ( -0.000000000000000000, 0.000000000000000000, 1.000000000000000000 ) ) ;
#6107=EDGE_CURVE ( 'NONE', #5434, #5227, #6003, .T. ) ;
#6126=DIRECTION ( 'NONE',  ( -1.000000000000000000, -0.000000000000000000, -0.000000000000000000 ) ) ;
#6143=ORIENTED_EDGE ( 'NONE', *, *, #6547, .T. ) ;
#6163=FACE_OUTER_BOUND ( 'NONE', #2897, .T. ) ;
#6183=DIRECTION ( 'NONE',  ( -0.000000000000000000, 1.000000000000000000, 0.000000000000000000 ) ) ;
#6197=DIRECTION ( 'NONE',  ( 1.000000000000000000, 0.000000000000000000, 0.000000000000000000 ) ) ;
#6214=ORIENTED_EDGE ( 'NONE', *, *, #660, .T. ) ;
#6216=DIRECTION ( 'NONE',  ( 0.000000000000000000, 0.000000000000000000, 1.000000000000000000 ) ) ;
#6225=ORIENTED_EDGE ( 'NONE', *, *, #1995, .T. ) ;
#6227=CARTESIAN_POINT ( 'NONE',  ( 0.000000000000000000, 0.000000000000000000, 140.0000000000000000 ) ) ;
#6229=FACE_OUTER_BOUND ( 'NONE', #7163, .T. ) ;
#6244=ORIENTED_EDGE ( 'NONE', *, *, #7160, .T. ) ;
#6280=AXIS2_PLACEMENT_3D ( 'NONE', #5136, #2860, #6335 ) ;
#6281=LINE ( 'NONE', #5716, #6945 ) ;
#6307=DIRECTION ( 'NONE',  ( 0.000000000000000000, -0.000000000000000000, -1.000000000000000000 ) ) ;
#6309=DIRECTION ( 'NONE',  ( -0.000000000000000000, -0.000000000000000000, -1.000000000000000000 ) ) ;
#6313=DIRECTION ( 'NONE',  ( 1.000000000000000000, 0.000000000000000000, -0.000000000000000000 ) ) ;
#6325=( LENGTH_UNIT ( ) NAMED_UNIT ( * ) SI_UNIT ( .MILLI., .METRE. ) );
#6326=APPLICATION_CONTEXT ( 'automotive_design' ) ;
#6335=DIRECTION ( 'NONE',  ( 0.000000000000000000, 0.000000000000000000, 1.000000000000000000 ) ) ;
#6351=EDGE_CURVE ( 'NONE', #3238, #1780, #5033, .T. ) ;
#6352=VERTEX_POINT ( 'NONE', #53 ) ;
#6358=LINE ( 'NONE', #1294, #3037 ) ;
#6363=ORIENTED_EDGE ( 'NONE', *, *, #6107, .F. ) ;
#6364=DIRECTION ( 'NONE',  ( 0.000000000000000000, 0.000000000000000000, 1.000000000000000000 ) ) ;
#6368=ADVANCED_FACE ( 'NONE', ( #3907 ), #1760, .F. ) ;
#6402=LINE ( 'NONE', #80, #6405 ) ;
#6403=ADVANCED_FACE ( 'NONE', ( #6229 ), #3471, .F. ) ;
#6405=VECTOR ( 'NONE', #221, 1000.000000000000000 ) ;
#6414=ORIENTED_EDGE ( 'NONE', *, *, #3232, .T. ) ;
#6432=ORIENTED_EDGE ( 'NONE', *, *, #3168, .T. ) ;
#6435=CARTESIAN_POINT ( 'NONE',  ( 4.999999999999993783, 8.660254037844390851, -140.0000000000000000 ) ) ;
#6439=ORIENTED_EDGE ( 'NONE', *, *, #1073, .T. ) ;
#6459=ORIENTED_EDGE ( 'NONE', *, *, #2636, .F. ) ;
#6464=( NAMED_UNIT ( * ) PLANE_ANGLE_UNIT ( ) SI_UNIT ( $, .RADIAN. ) );
#6472=STYLED_ITEM('',(#7432),#794);
#6481=CARTESIAN_POINT ( 'NONE',  ( 0.000000000000000000, 0.000000000000000000, 140.0000000000000000 ) ) ;
#6485=ORIENTED_EDGE ( 'NONE', *, *, #5366, .T. ) ;
#6492=DIRECTION ( 'NONE',  ( 1.000000000000000000, 0.000000000000000000, 0.000000000000000000 ) ) ;
#6528=CIRCLE ( 'NONE', #7002, 10.00000000000000000 ) ;
#6541=DIRECTION ( 'NONE',  ( 0.000000000000000000, 0.000000000000000000, 1.000000000000000000 ) ) ;
#6547=EDGE_CURVE ( 'NONE', #1550, #4157, #5315, .T. ) ;
#6567=FACE_OUTER_BOUND ( 'NONE', #4433, .T. ) ;
#6569=ORIENTED_EDGE ( 'NONE', *, *, #4171, .F. ) ;
#6613=EDGE_CURVE ( 'NONE', #1004, #7081, #5796, .T. ) ;
#6621=VECTOR ( 'NONE', #172, 1000.000000000000000 ) ;
#6623=AXIS2_PLACEMENT_3D ( 'NONE', #3167, #4398, #2700 ) ;
#6632=CARTESIAN_POINT ( 'NONE',  ( 0.000000000000000000, 0.000000000000000000, -140.0000000000000000 ) ) ;
#6649=DIRECTION ( 'NONE',  ( 0.000000000000000000, 0.000000000000000000, 1.000000000000000000 ) ) ;
#6666=PRODUCT_DEFINITION ( 'UNKNOWN', '', #3872, #6080 ) ;
#6722=MECHANICAL_DESIGN_GEOMETRIC_PRESENTATION_REPRESENTATION('',(#6472),#3911);
#6723=PLANE ( 'NONE',  #650 ) ;
#6734=EDGE_LOOP ( 'NONE', ( #476, #217, #942, #174 ) ) ;
#6735=VERTEX_POINT ( 'NONE', #424 ) ;
#6784=ORIENTED_EDGE ( 'NONE', *, *, #5085, .F. ) ;
#6814=VERTEX_POINT ( 'NONE', #3893 ) ;
#6828=EDGE_CURVE ( 'NONE', #2887, #5784, #5579, .T. ) ;
#6836=DIRECTION ( 'NONE',  ( -0.000000000000000000, -0.000000000000000000, -1.000000000000000000 ) ) ;
#6847=VERTEX_POINT ( 'NONE', #2856 ) ;
#6848=SHAPE_DEFINITION_REPRESENTATION ( #1342, #1193 ) ;
#6894=VERTEX_POINT ( 'NONE', #1994 ) ;
#6901=CARTESIAN_POINT ( 'NONE',  ( -5.000000000000000888, 8.660254037844390851, 150.0000000000000000 ) ) ;
#6908=CARTESIAN_POINT ( 'NONE',  ( 4.999999999999999112, -8.660254037844389075, 150.0000000000000000 ) ) ;
#6917=LINE ( 'NONE', #5120, #4811 ) ;
#6921=EDGE_LOOP ( 'NONE', ( #25, #4410, #2863, #6244 ) ) ;
#6942=DIRECTION ( 'NONE',  ( 0.000000000000000000, 0.000000000000000000, 1.000000000000000000 ) ) ;
#6945=VECTOR ( 'NONE', #5217, 1000.000000000000000 ) ;
#6952=DIRECTION ( 'NONE',  ( 1.000000000000000000, 0.000000000000000000, 0.000000000000000000 ) ) ;
#6961=AXIS2_PLACEMENT_3D ( 'NONE', #633, #5400, #2400 ) ;
#6967=EDGE_CURVE ( 'NONE', #5784, #2308, #6402, .T. ) ;
#6980=CARTESIAN_POINT ( 'NONE',  ( 0.000000000000000000, -8.660254037844389075, 140.0000000000000000 ) ) ;
#7002=AXIS2_PLACEMENT_3D ( 'NONE', #27, #2426, #1765 ) ;
#7005=EDGE_CURVE ( 'NONE', #3802, #6894, #634, .T. ) ;
#7015=VECTOR ( 'NONE', #4598, 1000.000000000000000 ) ;
#7022=CARTESIAN_POINT ( 'NONE',  ( 4.999999999999999112, -8.660254037844389075, 150.0000000000000000 ) ) ;
#7023=ORIENTED_EDGE ( 'NONE', *, *, #6828, .T. ) ;
#7034=DIRECTION ( 'NONE',  ( 0.000000000000000000, 0.000000000000000000, 1.000000000000000000 ) ) ;
#7062=UNCERTAINTY_MEASURE_WITH_UNIT (LENGTH_MEASURE( 1.000000000000000082E-05 ), #4138, 'distance_accuracy_value', 'NONE');
#7066=LINE ( 'NONE', #4475, #4440 ) ;
#7081=VERTEX_POINT ( 'NONE', #6435 ) ;
#7091=ORIENTED_EDGE ( 'NONE', *, *, #6351, .T. ) ;
#7140=CARTESIAN_POINT ( 'NONE',  ( -5.000000000000000888, 8.660254037844390851, 150.0000000000000000 ) ) ;
#7160=EDGE_CURVE ( 'NONE', #5784, #630, #2631, .T. ) ;
#7163=EDGE_LOOP ( 'NONE', ( #689, #4838 ) ) ;
#7199=PLANE ( 'NONE',  #4969 ) ;
#7202=CIRCLE ( 'NONE', #5524, 10.00000000000000000 ) ;
#7239=DIRECTION ( 'NONE',  ( -1.000000000000000000, 0.000000000000000000, 0.000000000000000000 ) ) ;
#7276=LINE ( 'NONE', #944, #4315 ) ;
#7278=DIRECTION ( 'NONE',  ( -0.000000000000000000, -0.000000000000000000, -1.000000000000000000 ) ) ;
#7285=ORIENTED_EDGE ( 'NONE', *, *, #5435, .T. ) ;
#7301=ORIENTED_EDGE ( 'NONE', *, *, #1641, .F. ) ;
#7303=DIRECTION ( 'NONE',  ( 0.000000000000000000, -0.000000000000000000, -1.000000000000000000 ) ) ;
#7310=CARTESIAN_POINT ( 'NONE',  ( 4.999999999999999112, -8.660254037844389075, 150.0000000000000000 ) ) ;
#7313=CARTESIAN_POINT ( 'NONE',  ( 0.000000000000000000, 0.000000000000000000, 140.0000000000000000 ) ) ;
#7316=VECTOR ( 'NONE', #6126, 1000.000000000000000 ) ;
#7322=FACE_OUTER_BOUND ( 'NONE', #4416, .T. ) ;
#7426=COLOUR_RGB('Sky Blue',0.24,0.69,0.87);
#7427=FILL_AREA_STYLE_COLOUR('',#7426);
#7428=FILL_AREA_STYLE('',(#7427));
#7429=SURFACE_STYLE_FILL_AREA(#7428);
#7430=SURFACE_SIDE_STYLE('',(#7429));
#7431=SURFACE_STYLE_USAGE(.BOTH.,#7430);
#7432=PRESENTATION_STYLE_ASSIGNMENT((#7431));
ENDSEC;
END-ISO-10303-21;
